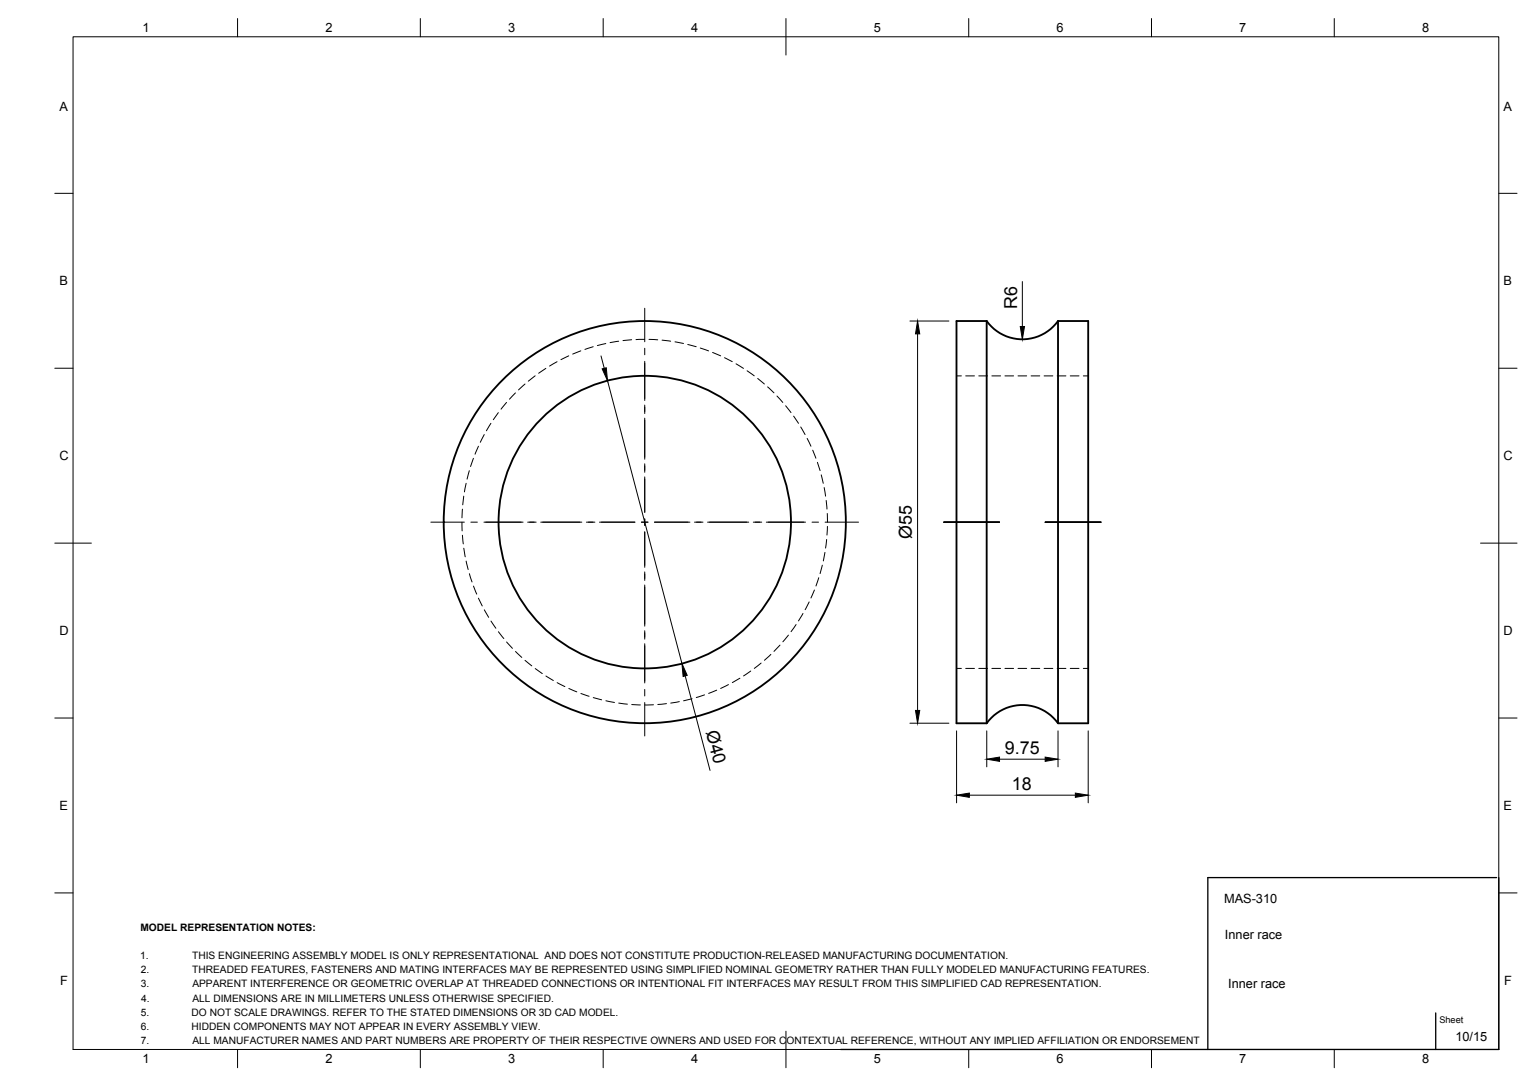
ISO-10303-21;
HEADER;
/* Generated by software containing ST-Developer
 * from STEP Tools, Inc. (www.steptools.com) 
 */

FILE_DESCRIPTION(
/* description */ ('Independent30mm screw-fed quill/spindle unit with16mm straight tool s
ocket, radial set screw, native reusable open ball bearings, retained 
inner/outer race stacks, keyed quill guide and M12x1.75 fine feed. Ext
ernal moving drive and tool not included. Ideal cage orbital links; in
dividual ball spin, force and preload not simulated. No drilling capac
ity, runout, speed, torque, load, life or machine safety rating.'),
/* implementation_level */ '2;1');

FILE_NAME(
/* name */ 'Inner race.step',
/* time_stamp */ '2026-11-08T18:59:42-08:00',
/* author */ (''),
/* organization */ (''),
/* preprocessor_version */ 'ST-DEVELOPER v20.2',
/* originating_system */ 'Autodesk Translation Framework v15.17.0.0',
/* authorisation */ '');

FILE_SCHEMA (('AUTOMOTIVE_DESIGN { 1 0 10303 214 3 1 1 }'));
ENDSEC;

DATA;
#10=MECHANICAL_DESIGN_GEOMETRIC_PRESENTATION_REPRESENTATION('',(#1604),#63898);
#236=TOROIDAL_SURFACE('',#16621,31.,6.);
#1568=SHAPE_REPRESENTATION_RELATIONSHIP('SRR','None',#64007,#1586);
#1586=ADVANCED_BREP_SHAPE_REPRESENTATION('',(#1622),#63892);
#1604=STYLED_ITEM('',(#64102),#1622);
#1622=MANIFOLD_SOLID_BREP('Body1',#15490);
#1706=FACE_BOUND('',#4327,.T.);
#1707=FACE_BOUND('',#4329,.T.);
#2335=CYLINDRICAL_SURFACE('',#16625,27.5);
#2336=CYLINDRICAL_SURFACE('',#16627,20.);
#2337=CYLINDRICAL_SURFACE('',#16630,27.5);
#2570=CIRCLE('',#16622,27.5);
#2571=CIRCLE('',#16623,6.);
#2572=CIRCLE('',#16624,27.5);
#2573=CIRCLE('',#16626,27.5);
#2574=CIRCLE('',#16628,20.);
#2575=CIRCLE('',#16629,20.);
#2576=CIRCLE('',#16631,27.5);
#3406=FACE_OUTER_BOUND('',#4322,.T.);
#3407=FACE_OUTER_BOUND('',#4323,.T.);
#3408=FACE_OUTER_BOUND('',#4324,.T.);
#3409=FACE_OUTER_BOUND('',#4325,.T.);
#3410=FACE_OUTER_BOUND('',#4326,.T.);
#3411=FACE_OUTER_BOUND('',#4328,.T.);
#4322=EDGE_LOOP('',(#13990,#13991,#13992,#13993));
#4323=EDGE_LOOP('',(#13994,#13995,#13996,#13997));
#4324=EDGE_LOOP('',(#13998,#13999,#14000,#14001));
#4325=EDGE_LOOP('',(#14002,#14003,#14004,#14005));
#4326=EDGE_LOOP('',(#14006));
#4327=EDGE_LOOP('',(#14007));
#4328=EDGE_LOOP('',(#14008));
#4329=EDGE_LOOP('',(#14009));
#5124=LINE('',#60388,#5887);
#5125=LINE('',#60394,#5888);
#5126=LINE('',#60399,#5889);
#5887=VECTOR('',#19422,27.5);
#5888=VECTOR('',#19429,20.);
#5889=VECTOR('',#19436,27.5);
#7330=VERTEX_POINT('',#60381);
#7331=VERTEX_POINT('',#60383);
#7332=VERTEX_POINT('',#60387);
#7333=VERTEX_POINT('',#60391);
#7334=VERTEX_POINT('',#60393);
#7335=VERTEX_POINT('',#60397);
#9584=EDGE_CURVE('',#7330,#7330,#2570,.T.);
#9585=EDGE_CURVE('',#7330,#7331,#2571,.T.);
#9586=EDGE_CURVE('',#7331,#7331,#2572,.T.);
#9587=EDGE_CURVE('',#7331,#7332,#5124,.T.);
#9588=EDGE_CURVE('',#7332,#7332,#2573,.T.);
#9589=EDGE_CURVE('',#7333,#7333,#2574,.T.);
#9590=EDGE_CURVE('',#7333,#7334,#5125,.T.);
#9591=EDGE_CURVE('',#7334,#7334,#2575,.T.);
#9592=EDGE_CURVE('',#7335,#7335,#2576,.T.);
#9593=EDGE_CURVE('',#7335,#7330,#5126,.T.);
#13990=ORIENTED_EDGE('',*,*,#9584,.F.);
#13991=ORIENTED_EDGE('',*,*,#9585,.T.);
#13992=ORIENTED_EDGE('',*,*,#9586,.F.);
#13993=ORIENTED_EDGE('',*,*,#9585,.F.);
#13994=ORIENTED_EDGE('',*,*,#9586,.T.);
#13995=ORIENTED_EDGE('',*,*,#9587,.T.);
#13996=ORIENTED_EDGE('',*,*,#9588,.T.);
#13997=ORIENTED_EDGE('',*,*,#9587,.F.);
#13998=ORIENTED_EDGE('',*,*,#9589,.F.);
#13999=ORIENTED_EDGE('',*,*,#9590,.T.);
#14000=ORIENTED_EDGE('',*,*,#9591,.T.);
#14001=ORIENTED_EDGE('',*,*,#9590,.F.);
#14002=ORIENTED_EDGE('',*,*,#9592,.F.);
#14003=ORIENTED_EDGE('',*,*,#9593,.T.);
#14004=ORIENTED_EDGE('',*,*,#9584,.T.);
#14005=ORIENTED_EDGE('',*,*,#9593,.F.);
#14006=ORIENTED_EDGE('',*,*,#9592,.T.);
#14007=ORIENTED_EDGE('',*,*,#9589,.T.);
#14008=ORIENTED_EDGE('',*,*,#9588,.F.);
#14009=ORIENTED_EDGE('',*,*,#9591,.F.);
#14611=PLANE('',#16632);
#14612=PLANE('',#16633);
#15386=ADVANCED_FACE('',(#3406),#236,.F.);
#15387=ADVANCED_FACE('',(#3407),#2335,.T.);
#15388=ADVANCED_FACE('',(#3408),#2336,.F.);
#15389=ADVANCED_FACE('',(#3409),#2337,.T.);
#15390=ADVANCED_FACE('',(#3410,#1706),#14611,.T.);
#15391=ADVANCED_FACE('',(#3411,#1707),#14612,.F.);
#15490=CLOSED_SHELL('',(#15386,#15387,#15388,#15389,#15390,#15391));
#16620=AXIS2_PLACEMENT_3D('',#60379,#19410,#19411);
#16621=AXIS2_PLACEMENT_3D('',#60380,#19412,#19413);
#16622=AXIS2_PLACEMENT_3D('',#60382,#19414,#19415);
#16623=AXIS2_PLACEMENT_3D('',#60384,#19416,#19417);
#16624=AXIS2_PLACEMENT_3D('',#60385,#19418,#19419);
#16625=AXIS2_PLACEMENT_3D('',#60386,#19420,#19421);
#16626=AXIS2_PLACEMENT_3D('',#60389,#19423,#19424);
#16627=AXIS2_PLACEMENT_3D('',#60390,#19425,#19426);
#16628=AXIS2_PLACEMENT_3D('',#60392,#19427,#19428);
#16629=AXIS2_PLACEMENT_3D('',#60395,#19430,#19431);
#16630=AXIS2_PLACEMENT_3D('',#60396,#19432,#19433);
#16631=AXIS2_PLACEMENT_3D('',#60398,#19434,#19435);
#16632=AXIS2_PLACEMENT_3D('',#60400,#19437,#19438);
#16633=AXIS2_PLACEMENT_3D('',#60401,#19439,#19440);
#19410=DIRECTION('axis',(0.,0.,1.));
#19411=DIRECTION('refdir',(1.,0.,0.));
#19412=DIRECTION('center_axis',(0.,0.,1.));
#19413=DIRECTION('ref_axis',(1.,0.,0.));
#19414=DIRECTION('center_axis',(0.,0.,1.));
#19415=DIRECTION('ref_axis',(1.,0.,0.));
#19416=DIRECTION('center_axis',(-1.22464679914735E-16,1.,0.));
#19417=DIRECTION('ref_axis',(-1.,-1.22464679914735E-16,0.));
#19418=DIRECTION('center_axis',(0.,0.,-1.));
#19419=DIRECTION('ref_axis',(1.,0.,0.));
#19420=DIRECTION('center_axis',(0.,0.,1.));
#19421=DIRECTION('ref_axis',(1.,0.,0.));
#19422=DIRECTION('',(0.,0.,-1.));
#19423=DIRECTION('center_axis',(0.,0.,1.));
#19424=DIRECTION('ref_axis',(1.,0.,0.));
#19425=DIRECTION('center_axis',(0.,0.,1.));
#19426=DIRECTION('ref_axis',(1.,0.,0.));
#19427=DIRECTION('center_axis',(0.,0.,-1.));
#19428=DIRECTION('ref_axis',(1.,0.,0.));
#19429=DIRECTION('',(0.,0.,-1.));
#19430=DIRECTION('center_axis',(0.,0.,-1.));
#19431=DIRECTION('ref_axis',(1.,0.,0.));
#19432=DIRECTION('center_axis',(0.,0.,1.));
#19433=DIRECTION('ref_axis',(1.,0.,0.));
#19434=DIRECTION('center_axis',(0.,0.,1.));
#19435=DIRECTION('ref_axis',(1.,0.,0.));
#19436=DIRECTION('',(0.,0.,-1.));
#19437=DIRECTION('center_axis',(0.,0.,1.));
#19438=DIRECTION('ref_axis',(1.,0.,0.));
#19439=DIRECTION('center_axis',(0.,0.,1.));
#19440=DIRECTION('ref_axis',(1.,0.,0.));
#60379=CARTESIAN_POINT('',(0.,0.,0.));
#60380=CARTESIAN_POINT('Origin',(0.,0.,0.));
#60381=CARTESIAN_POINT('',(-27.5,-3.36777869765522E-15,4.87339717240448));
#60382=CARTESIAN_POINT('Origin',(0.,0.,4.87339717240448));
#60383=CARTESIAN_POINT('',(-27.5,3.36777869765522E-15,-4.87339717240448));
#60384=CARTESIAN_POINT('Origin',(-31.,-3.7964050773568E-15,0.));
#60385=CARTESIAN_POINT('Origin',(0.,0.,-4.87339717240448));
#60386=CARTESIAN_POINT('Origin',(0.,0.,-9.));
#60387=CARTESIAN_POINT('',(-27.5,-3.36777869765522E-15,-9.));
#60388=CARTESIAN_POINT('',(-27.5,-3.36777869765522E-15,-9.));
#60389=CARTESIAN_POINT('Origin',(0.,0.,-9.));
#60390=CARTESIAN_POINT('Origin',(0.,0.,-9.));
#60391=CARTESIAN_POINT('',(-20.,-2.44929359829471E-15,9.));
#60392=CARTESIAN_POINT('Origin',(0.,0.,9.));
#60393=CARTESIAN_POINT('',(-20.,-2.44929359829471E-15,-9.));
#60394=CARTESIAN_POINT('',(-20.,-2.44929359829471E-15,-9.));
#60395=CARTESIAN_POINT('Origin',(0.,0.,-9.));
#60396=CARTESIAN_POINT('Origin',(0.,0.,-9.));
#60397=CARTESIAN_POINT('',(-27.5,-3.36777869765522E-15,9.));
#60398=CARTESIAN_POINT('Origin',(0.,0.,9.));
#60399=CARTESIAN_POINT('',(-27.5,-3.36777869765522E-15,-9.));
#60400=CARTESIAN_POINT('Origin',(0.,0.,9.));
#60401=CARTESIAN_POINT('Origin',(0.,0.,-9.));
#63872=UNCERTAINTY_MEASURE_WITH_UNIT(LENGTH_MEASURE(0.01),#63899,
'DISTANCE_ACCURACY_VALUE',
'Maximum model space distance between geometric entities at asserted c
onnectivities');
#63878=UNCERTAINTY_MEASURE_WITH_UNIT(LENGTH_MEASURE(0.01),#63899,
'DISTANCE_ACCURACY_VALUE',
'Maximum model space distance between geometric entities at asserted c
onnectivities');
#63892=(
GEOMETRIC_REPRESENTATION_CONTEXT(3)
GLOBAL_UNCERTAINTY_ASSIGNED_CONTEXT((#63872))
GLOBAL_UNIT_ASSIGNED_CONTEXT((#63899,#63901,#63902))
REPRESENTATION_CONTEXT('','3D')
);
#63898=(
GEOMETRIC_REPRESENTATION_CONTEXT(3)
GLOBAL_UNCERTAINTY_ASSIGNED_CONTEXT((#63878))
GLOBAL_UNIT_ASSIGNED_CONTEXT((#63899,#63901,#63902))
REPRESENTATION_CONTEXT('','3D')
);
#63899=(
LENGTH_UNIT()
NAMED_UNIT(*)
SI_UNIT(.MILLI.,.METRE.)
);
#63901=(
NAMED_UNIT(*)
PLANE_ANGLE_UNIT()
SI_UNIT($,.RADIAN.)
);
#63902=(
NAMED_UNIT(*)
SI_UNIT($,.STERADIAN.)
SOLID_ANGLE_UNIT()
);
#63916=SHAPE_DEFINITION_REPRESENTATION(#63935,#64007);
#63935=PRODUCT_DEFINITION_SHAPE('',$,#64027);
#64007=SHAPE_REPRESENTATION('',(#16620),#63892);
#64013=PRODUCT_DEFINITION_CONTEXT('part definition',#64072,'design');
#64027=PRODUCT_DEFINITION('Inner race','Inner race',#64046,#64013);
#64046=PRODUCT_DEFINITION_FORMATION('',$,#64087);
#64072=APPLICATION_CONTEXT(
'Core Data for Automotive Mechanical Design Process');
#64073=PRODUCT_CONTEXT('part definition',#64072,'mechanical');
#64087=PRODUCT('Inner race','Inner race',$,(#64073));
#64102=PRESENTATION_STYLE_ASSIGNMENT((#64115));
#64115=SURFACE_STYLE_USAGE(.BOTH.,#64128);
#64128=SURFACE_SIDE_STYLE('',(#64141));
#64141=SURFACE_STYLE_FILL_AREA(#64154);
#64154=FILL_AREA_STYLE('Inner race gray',(#64167));
#64167=FILL_AREA_STYLE_COLOUR('Inner race gray',#64180);
#64180=COLOUR_RGB('Inner race gray',0.576470588235294,0.615686274509804,
0.666666666666667);
ENDSEC;
END-ISO-10303-21;
